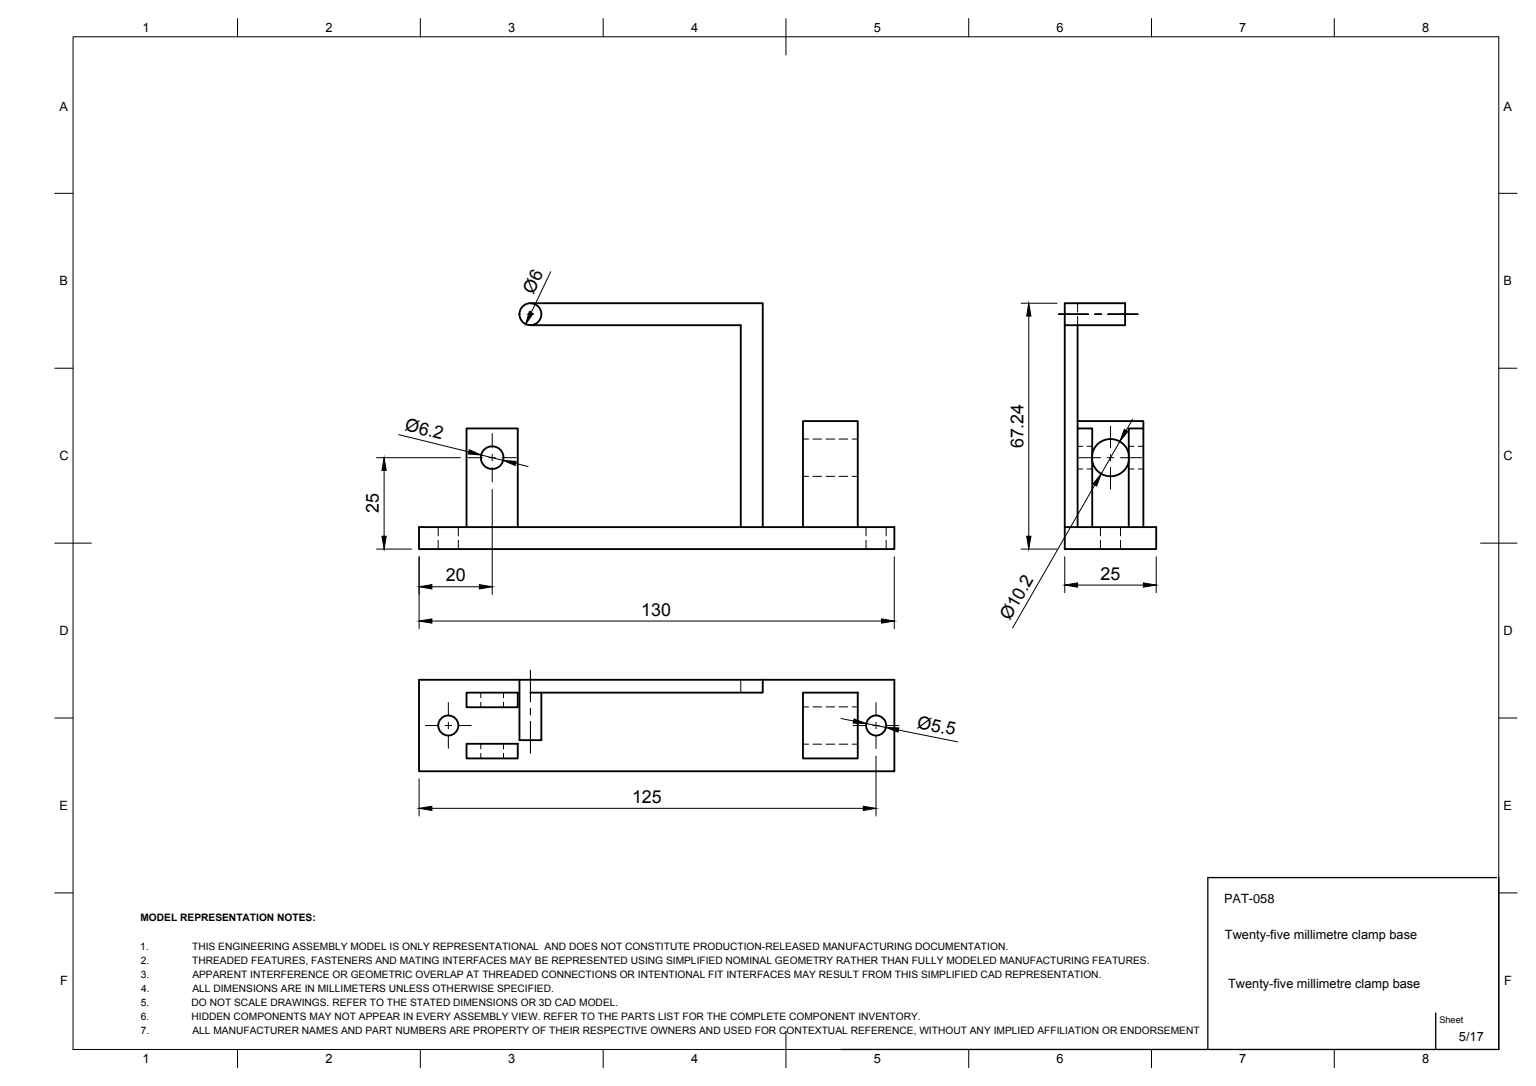
ISO-10303-21;
HEADER;
/* Generated by software containing ST-Developer
 * from STEP Tools, Inc. (www.steptools.com) 
 */

FILE_DESCRIPTION(
/* description */ ('Horizontal push-pull toggle clamp'),
/* implementation_level */ '2;1');

FILE_NAME(
/* name */ 'Twenty-five millimetre clamp base.step',
/* time_stamp */ '2026-10-27T21:21:09-07:00',
/* author */ (''),
/* organization */ (''),
/* preprocessor_version */ 'ST-DEVELOPER v20.2',
/* originating_system */ 'Autodesk Translation Framework v15.17.0.0',
/* authorisation */ '');

FILE_SCHEMA (('AUTOMOTIVE_DESIGN { 1 0 10303 214 3 1 1 }'));
ENDSEC;

DATA;
#10=MECHANICAL_DESIGN_GEOMETRIC_PRESENTATION_REPRESENTATION('',(#185),#4791);
#159=SHAPE_REPRESENTATION_RELATIONSHIP('SRR','None',#4862,#172);
#172=ADVANCED_BREP_SHAPE_REPRESENTATION('',(#198),#4775);
#185=STYLED_ITEM('',(#5002),#198);
#198=MANIFOLD_SOLID_BREP('Body1',#2629);
#210=FACE_BOUND('',#522,.T.);
#211=FACE_BOUND('',#523,.T.);
#212=FACE_BOUND('',#524,.T.);
#213=FACE_BOUND('',#525,.T.);
#214=FACE_BOUND('',#526,.T.);
#215=FACE_BOUND('',#532,.T.);
#216=FACE_BOUND('',#534,.T.);
#217=FACE_BOUND('',#540,.T.);
#218=FACE_BOUND('',#545,.T.);
#219=FACE_BOUND('',#547,.T.);
#220=FACE_BOUND('',#552,.T.);
#221=FACE_BOUND('',#557,.T.);
#222=FACE_BOUND('',#558,.T.);
#256=PLANE('',#2795);
#257=PLANE('',#2796);
#258=PLANE('',#2797);
#259=PLANE('',#2798);
#260=PLANE('',#2799);
#261=PLANE('',#2800);
#262=PLANE('',#2801);
#263=PLANE('',#2802);
#264=PLANE('',#2812);
#265=PLANE('',#2813);
#266=PLANE('',#2814);
#267=PLANE('',#2815);
#268=PLANE('',#2816);
#269=PLANE('',#2823);
#270=PLANE('',#2824);
#271=PLANE('',#2825);
#272=PLANE('',#2826);
#273=PLANE('',#2827);
#274=PLANE('',#2828);
#275=PLANE('',#2829);
#276=PLANE('',#2830);
#277=PLANE('',#2831);
#278=PLANE('',#2832);
#279=PLANE('',#2833);
#280=PLANE('',#2834);
#281=PLANE('',#2835);
#282=PLANE('',#2836);
#362=FACE_OUTER_BOUND('',#513,.T.);
#363=FACE_OUTER_BOUND('',#514,.T.);
#364=FACE_OUTER_BOUND('',#515,.T.);
#365=FACE_OUTER_BOUND('',#516,.T.);
#366=FACE_OUTER_BOUND('',#517,.T.);
#367=FACE_OUTER_BOUND('',#518,.T.);
#368=FACE_OUTER_BOUND('',#519,.T.);
#369=FACE_OUTER_BOUND('',#520,.T.);
#370=FACE_OUTER_BOUND('',#521,.T.);
#371=FACE_OUTER_BOUND('',#527,.T.);
#372=FACE_OUTER_BOUND('',#528,.T.);
#373=FACE_OUTER_BOUND('',#529,.T.);
#374=FACE_OUTER_BOUND('',#530,.T.);
#375=FACE_OUTER_BOUND('',#531,.T.);
#376=FACE_OUTER_BOUND('',#533,.T.);
#377=FACE_OUTER_BOUND('',#535,.T.);
#378=FACE_OUTER_BOUND('',#536,.T.);
#379=FACE_OUTER_BOUND('',#537,.T.);
#380=FACE_OUTER_BOUND('',#538,.T.);
#381=FACE_OUTER_BOUND('',#539,.T.);
#382=FACE_OUTER_BOUND('',#541,.T.);
#383=FACE_OUTER_BOUND('',#542,.T.);
#384=FACE_OUTER_BOUND('',#543,.T.);
#385=FACE_OUTER_BOUND('',#544,.T.);
#386=FACE_OUTER_BOUND('',#546,.T.);
#387=FACE_OUTER_BOUND('',#548,.T.);
#388=FACE_OUTER_BOUND('',#549,.T.);
#389=FACE_OUTER_BOUND('',#550,.T.);
#390=FACE_OUTER_BOUND('',#551,.T.);
#391=FACE_OUTER_BOUND('',#553,.T.);
#392=FACE_OUTER_BOUND('',#554,.T.);
#393=FACE_OUTER_BOUND('',#555,.T.);
#394=FACE_OUTER_BOUND('',#556,.T.);
#513=EDGE_LOOP('',(#1783,#1784,#1785,#1786,#1787,#1788,#1789,#1790));
#514=EDGE_LOOP('',(#1791));
#515=EDGE_LOOP('',(#1792,#1793,#1794,#1795,#1796,#1797,#1798,#1799,#1800,
#1801,#1802));
#516=EDGE_LOOP('',(#1803,#1804,#1805,#1806));
#517=EDGE_LOOP('',(#1807,#1808,#1809,#1810));
#518=EDGE_LOOP('',(#1811,#1812,#1813,#1814));
#519=EDGE_LOOP('',(#1815,#1816,#1817,#1818));
#520=EDGE_LOOP('',(#1819,#1820,#1821,#1822,#1823,#1824));
#521=EDGE_LOOP('',(#1825,#1826,#1827,#1828,#1829,#1830,#1831,#1832));
#522=EDGE_LOOP('',(#1833,#1834,#1835,#1836));
#523=EDGE_LOOP('',(#1837,#1838,#1839,#1840));
#524=EDGE_LOOP('',(#1841,#1842,#1843,#1844));
#525=EDGE_LOOP('',(#1845));
#526=EDGE_LOOP('',(#1846));
#527=EDGE_LOOP('',(#1847,#1848,#1849,#1850));
#528=EDGE_LOOP('',(#1851,#1852,#1853,#1854));
#529=EDGE_LOOP('',(#1855,#1856,#1857,#1858));
#530=EDGE_LOOP('',(#1859,#1860,#1861,#1862));
#531=EDGE_LOOP('',(#1863,#1864,#1865,#1866));
#532=EDGE_LOOP('',(#1867));
#533=EDGE_LOOP('',(#1868,#1869,#1870,#1871));
#534=EDGE_LOOP('',(#1872));
#535=EDGE_LOOP('',(#1873,#1874,#1875,#1876));
#536=EDGE_LOOP('',(#1877,#1878,#1879,#1880));
#537=EDGE_LOOP('',(#1881,#1882,#1883,#1884));
#538=EDGE_LOOP('',(#1885,#1886,#1887,#1888));
#539=EDGE_LOOP('',(#1889,#1890,#1891,#1892));
#540=EDGE_LOOP('',(#1893));
#541=EDGE_LOOP('',(#1894,#1895,#1896,#1897));
#542=EDGE_LOOP('',(#1898,#1899,#1900,#1901));
#543=EDGE_LOOP('',(#1902,#1903,#1904,#1905));
#544=EDGE_LOOP('',(#1906,#1907,#1908,#1909));
#545=EDGE_LOOP('',(#1910));
#546=EDGE_LOOP('',(#1911,#1912,#1913,#1914));
#547=EDGE_LOOP('',(#1915));
#548=EDGE_LOOP('',(#1916,#1917,#1918,#1919));
#549=EDGE_LOOP('',(#1920,#1921,#1922,#1923));
#550=EDGE_LOOP('',(#1924,#1925,#1926,#1927));
#551=EDGE_LOOP('',(#1928,#1929,#1930,#1931));
#552=EDGE_LOOP('',(#1932));
#553=EDGE_LOOP('',(#1933,#1934,#1935,#1936));
#554=EDGE_LOOP('',(#1937,#1938,#1939,#1940));
#555=EDGE_LOOP('',(#1941,#1942,#1943,#1944));
#556=EDGE_LOOP('',(#1945,#1946,#1947,#1948));
#557=EDGE_LOOP('',(#1949));
#558=EDGE_LOOP('',(#1950));
#710=CIRCLE('',#2791,0.3);
#711=CIRCLE('',#2792,0.3);
#712=CIRCLE('',#2793,0.3);
#713=CIRCLE('',#2794,0.3);
#714=CIRCLE('',#2803,0.275);
#715=CIRCLE('',#2804,0.275);
#716=CIRCLE('',#2806,0.275);
#717=CIRCLE('',#2808,0.275);
#718=CIRCLE('',#2810,0.51);
#719=CIRCLE('',#2811,0.51);
#720=CIRCLE('',#2818,0.31);
#721=CIRCLE('',#2819,0.31);
#722=CIRCLE('',#2821,0.31);
#723=CIRCLE('',#2822,0.31);
#796=LINE('',#3862,#1016);
#797=LINE('',#3866,#1017);
#798=LINE('',#3870,#1018);
#799=LINE('',#3876,#1019);
#800=LINE('',#3878,#1020);
#801=LINE('',#3880,#1021);
#802=LINE('',#3882,#1022);
#803=LINE('',#3884,#1023);
#804=LINE('',#3886,#1024);
#805=LINE('',#3888,#1025);
#806=LINE('',#3890,#1026);
#807=LINE('',#3891,#1027);
#808=LINE('',#3894,#1028);
#809=LINE('',#3895,#1029);
#810=LINE('',#3898,#1030);
#811=LINE('',#3899,#1031);
#812=LINE('',#3902,#1032);
#813=LINE('',#3903,#1033);
#814=LINE('',#3906,#1034);
#815=LINE('',#3907,#1035);
#816=LINE('',#3909,#1036);
#817=LINE('',#3912,#1037);
#818=LINE('',#3914,#1038);
#819=LINE('',#3915,#1039);
#820=LINE('',#3918,#1040);
#821=LINE('',#3920,#1041);
#822=LINE('',#3922,#1042);
#823=LINE('',#3923,#1043);
#824=LINE('',#3926,#1044);
#825=LINE('',#3928,#1045);
#826=LINE('',#3930,#1046);
#827=LINE('',#3931,#1047);
#828=LINE('',#3934,#1048);
#829=LINE('',#3936,#1049);
#830=LINE('',#3938,#1050);
#831=LINE('',#3939,#1051);
#832=LINE('',#3947,#1052);
#833=LINE('',#3951,#1053);
#834=LINE('',#3956,#1054);
#835=LINE('',#3960,#1055);
#836=LINE('',#3962,#1056);
#837=LINE('',#3963,#1057);
#838=LINE('',#3966,#1058);
#839=LINE('',#3967,#1059);
#840=LINE('',#3970,#1060);
#841=LINE('',#3971,#1061);
#842=LINE('',#3973,#1062);
#843=LINE('',#3979,#1063);
#844=LINE('',#3985,#1064);
#845=LINE('',#3989,#1065);
#846=LINE('',#3991,#1066);
#847=LINE('',#3992,#1067);
#848=LINE('',#3995,#1068);
#849=LINE('',#3996,#1069);
#850=LINE('',#3999,#1070);
#851=LINE('',#4000,#1071);
#852=LINE('',#4002,#1072);
#853=LINE('',#4006,#1073);
#854=LINE('',#4008,#1074);
#855=LINE('',#4009,#1075);
#856=LINE('',#4012,#1076);
#857=LINE('',#4013,#1077);
#858=LINE('',#4016,#1078);
#859=LINE('',#4017,#1079);
#860=LINE('',#4019,#1080);
#861=LINE('',#4023,#1081);
#862=LINE('',#4024,#1082);
#863=LINE('',#4027,#1083);
#864=LINE('',#4028,#1084);
#865=LINE('',#4030,#1085);
#1016=VECTOR('',#3078,1.);
#1017=VECTOR('',#3081,1.);
#1018=VECTOR('',#3084,0.3);
#1019=VECTOR('',#3093,1.);
#1020=VECTOR('',#3094,1.);
#1021=VECTOR('',#3095,1.);
#1022=VECTOR('',#3096,1.);
#1023=VECTOR('',#3097,1.);
#1024=VECTOR('',#3098,1.);
#1025=VECTOR('',#3099,1.);
#1026=VECTOR('',#3100,1.);
#1027=VECTOR('',#3101,1.);
#1028=VECTOR('',#3104,1.);
#1029=VECTOR('',#3105,1.);
#1030=VECTOR('',#3108,1.);
#1031=VECTOR('',#3109,1.);
#1032=VECTOR('',#3112,1.);
#1033=VECTOR('',#3113,1.);
#1034=VECTOR('',#3116,1.);
#1035=VECTOR('',#3117,1.);
#1036=VECTOR('',#3120,1.);
#1037=VECTOR('',#3123,1.);
#1038=VECTOR('',#3124,1.);
#1039=VECTOR('',#3125,1.);
#1040=VECTOR('',#3126,1.);
#1041=VECTOR('',#3127,1.);
#1042=VECTOR('',#3128,1.);
#1043=VECTOR('',#3129,1.);
#1044=VECTOR('',#3130,1.);
#1045=VECTOR('',#3131,1.);
#1046=VECTOR('',#3132,1.);
#1047=VECTOR('',#3133,1.);
#1048=VECTOR('',#3134,1.);
#1049=VECTOR('',#3135,1.);
#1050=VECTOR('',#3136,1.);
#1051=VECTOR('',#3137,1.);
#1052=VECTOR('',#3146,0.275);
#1053=VECTOR('',#3151,0.275);
#1054=VECTOR('',#3156,0.51);
#1055=VECTOR('',#3161,1.);
#1056=VECTOR('',#3162,1.);
#1057=VECTOR('',#3163,1.);
#1058=VECTOR('',#3166,1.);
#1059=VECTOR('',#3167,1.);
#1060=VECTOR('',#3170,1.);
#1061=VECTOR('',#3171,1.);
#1062=VECTOR('',#3174,1.);
#1063=VECTOR('',#3181,0.31);
#1064=VECTOR('',#3188,0.31);
#1065=VECTOR('',#3193,1.);
#1066=VECTOR('',#3194,1.);
#1067=VECTOR('',#3195,1.);
#1068=VECTOR('',#3198,1.);
#1069=VECTOR('',#3199,1.);
#1070=VECTOR('',#3202,1.);
#1071=VECTOR('',#3203,1.);
#1072=VECTOR('',#3206,1.);
#1073=VECTOR('',#3211,1.);
#1074=VECTOR('',#3212,1.);
#1075=VECTOR('',#3213,1.);
#1076=VECTOR('',#3216,1.);
#1077=VECTOR('',#3217,1.);
#1078=VECTOR('',#3220,1.);
#1079=VECTOR('',#3221,1.);
#1080=VECTOR('',#3224,1.);
#1081=VECTOR('',#3229,1.);
#1082=VECTOR('',#3230,1.);
#1083=VECTOR('',#3233,1.);
#1084=VECTOR('',#3234,1.);
#1085=VECTOR('',#3237,1.);
#1236=VERTEX_POINT('',#3860);
#1237=VERTEX_POINT('',#3861);
#1238=VERTEX_POINT('',#3863);
#1239=VERTEX_POINT('',#3865);
#1240=VERTEX_POINT('',#3867);
#1241=VERTEX_POINT('',#3869);
#1242=VERTEX_POINT('',#3875);
#1243=VERTEX_POINT('',#3877);
#1244=VERTEX_POINT('',#3879);
#1245=VERTEX_POINT('',#3881);
#1246=VERTEX_POINT('',#3883);
#1247=VERTEX_POINT('',#3885);
#1248=VERTEX_POINT('',#3887);
#1249=VERTEX_POINT('',#3889);
#1250=VERTEX_POINT('',#3893);
#1251=VERTEX_POINT('',#3897);
#1252=VERTEX_POINT('',#3901);
#1253=VERTEX_POINT('',#3905);
#1254=VERTEX_POINT('',#3911);
#1255=VERTEX_POINT('',#3913);
#1256=VERTEX_POINT('',#3916);
#1257=VERTEX_POINT('',#3917);
#1258=VERTEX_POINT('',#3919);
#1259=VERTEX_POINT('',#3921);
#1260=VERTEX_POINT('',#3924);
#1261=VERTEX_POINT('',#3925);
#1262=VERTEX_POINT('',#3927);
#1263=VERTEX_POINT('',#3929);
#1264=VERTEX_POINT('',#3932);
#1265=VERTEX_POINT('',#3933);
#1266=VERTEX_POINT('',#3935);
#1267=VERTEX_POINT('',#3937);
#1268=VERTEX_POINT('',#3940);
#1269=VERTEX_POINT('',#3942);
#1270=VERTEX_POINT('',#3945);
#1271=VERTEX_POINT('',#3949);
#1272=VERTEX_POINT('',#3953);
#1273=VERTEX_POINT('',#3955);
#1274=VERTEX_POINT('',#3959);
#1275=VERTEX_POINT('',#3961);
#1276=VERTEX_POINT('',#3965);
#1277=VERTEX_POINT('',#3969);
#1278=VERTEX_POINT('',#3976);
#1279=VERTEX_POINT('',#3978);
#1280=VERTEX_POINT('',#3982);
#1281=VERTEX_POINT('',#3984);
#1282=VERTEX_POINT('',#3988);
#1283=VERTEX_POINT('',#3990);
#1284=VERTEX_POINT('',#3994);
#1285=VERTEX_POINT('',#3998);
#1286=VERTEX_POINT('',#4005);
#1287=VERTEX_POINT('',#4007);
#1288=VERTEX_POINT('',#4011);
#1289=VERTEX_POINT('',#4015);
#1290=VERTEX_POINT('',#4022);
#1291=VERTEX_POINT('',#4026);
#1453=EDGE_CURVE('',#1236,#1237,#796,.T.);
#1454=EDGE_CURVE('',#1238,#1236,#710,.T.);
#1455=EDGE_CURVE('',#1238,#1239,#797,.T.);
#1456=EDGE_CURVE('',#1240,#1239,#711,.T.);
#1457=EDGE_CURVE('',#1240,#1241,#798,.T.);
#1458=EDGE_CURVE('',#1241,#1241,#712,.T.);
#1459=EDGE_CURVE('',#1237,#1240,#713,.T.);
#1460=EDGE_CURVE('',#1239,#1242,#799,.T.);
#1461=EDGE_CURVE('',#1242,#1243,#800,.T.);
#1462=EDGE_CURVE('',#1244,#1243,#801,.T.);
#1463=EDGE_CURVE('',#1245,#1244,#802,.T.);
#1464=EDGE_CURVE('',#1245,#1246,#803,.T.);
#1465=EDGE_CURVE('',#1246,#1247,#804,.T.);
#1466=EDGE_CURVE('',#1248,#1247,#805,.T.);
#1467=EDGE_CURVE('',#1248,#1249,#806,.T.);
#1468=EDGE_CURVE('',#1249,#1237,#807,.T.);
#1469=EDGE_CURVE('',#1250,#1249,#808,.T.);
#1470=EDGE_CURVE('',#1236,#1250,#809,.T.);
#1471=EDGE_CURVE('',#1251,#1238,#810,.T.);
#1472=EDGE_CURVE('',#1251,#1242,#811,.T.);
#1473=EDGE_CURVE('',#1252,#1251,#812,.T.);
#1474=EDGE_CURVE('',#1243,#1252,#813,.T.);
#1475=EDGE_CURVE('',#1253,#1248,#814,.T.);
#1476=EDGE_CURVE('',#1250,#1253,#815,.T.);
#1477=EDGE_CURVE('',#1252,#1253,#816,.T.);
#1478=EDGE_CURVE('',#1247,#1254,#817,.T.);
#1479=EDGE_CURVE('',#1254,#1255,#818,.T.);
#1480=EDGE_CURVE('',#1255,#1244,#819,.T.);
#1481=EDGE_CURVE('',#1256,#1257,#820,.T.);
#1482=EDGE_CURVE('',#1257,#1258,#821,.T.);
#1483=EDGE_CURVE('',#1258,#1259,#822,.T.);
#1484=EDGE_CURVE('',#1259,#1256,#823,.T.);
#1485=EDGE_CURVE('',#1260,#1261,#824,.T.);
#1486=EDGE_CURVE('',#1261,#1262,#825,.T.);
#1487=EDGE_CURVE('',#1262,#1263,#826,.T.);
#1488=EDGE_CURVE('',#1263,#1260,#827,.T.);
#1489=EDGE_CURVE('',#1264,#1265,#828,.T.);
#1490=EDGE_CURVE('',#1265,#1266,#829,.T.);
#1491=EDGE_CURVE('',#1266,#1267,#830,.T.);
#1492=EDGE_CURVE('',#1267,#1264,#831,.T.);
#1493=EDGE_CURVE('',#1268,#1268,#714,.T.);
#1494=EDGE_CURVE('',#1269,#1269,#715,.T.);
#1495=EDGE_CURVE('',#1270,#1270,#716,.T.);
#1496=EDGE_CURVE('',#1270,#1269,#832,.T.);
#1497=EDGE_CURVE('',#1271,#1271,#717,.T.);
#1498=EDGE_CURVE('',#1271,#1268,#833,.T.);
#1499=EDGE_CURVE('',#1272,#1272,#718,.T.);
#1500=EDGE_CURVE('',#1272,#1273,#834,.T.);
#1501=EDGE_CURVE('',#1273,#1273,#719,.T.);
#1502=EDGE_CURVE('',#1265,#1274,#835,.T.);
#1503=EDGE_CURVE('',#1274,#1275,#836,.T.);
#1504=EDGE_CURVE('',#1275,#1266,#837,.T.);
#1505=EDGE_CURVE('',#1276,#1264,#838,.T.);
#1506=EDGE_CURVE('',#1274,#1276,#839,.T.);
#1507=EDGE_CURVE('',#1275,#1277,#840,.T.);
#1508=EDGE_CURVE('',#1267,#1277,#841,.T.);
#1509=EDGE_CURVE('',#1277,#1276,#842,.T.);
#1510=EDGE_CURVE('',#1278,#1278,#720,.T.);
#1511=EDGE_CURVE('',#1278,#1279,#843,.T.);
#1512=EDGE_CURVE('',#1279,#1279,#721,.T.);
#1513=EDGE_CURVE('',#1280,#1280,#722,.T.);
#1514=EDGE_CURVE('',#1280,#1281,#844,.T.);
#1515=EDGE_CURVE('',#1281,#1281,#723,.T.);
#1516=EDGE_CURVE('',#1261,#1282,#845,.T.);
#1517=EDGE_CURVE('',#1282,#1283,#846,.T.);
#1518=EDGE_CURVE('',#1283,#1262,#847,.T.);
#1519=EDGE_CURVE('',#1284,#1260,#848,.T.);
#1520=EDGE_CURVE('',#1282,#1284,#849,.T.);
#1521=EDGE_CURVE('',#1283,#1285,#850,.T.);
#1522=EDGE_CURVE('',#1263,#1285,#851,.T.);
#1523=EDGE_CURVE('',#1285,#1284,#852,.T.);
#1524=EDGE_CURVE('',#1257,#1286,#853,.T.);
#1525=EDGE_CURVE('',#1286,#1287,#854,.T.);
#1526=EDGE_CURVE('',#1287,#1258,#855,.T.);
#1527=EDGE_CURVE('',#1288,#1256,#856,.T.);
#1528=EDGE_CURVE('',#1286,#1288,#857,.T.);
#1529=EDGE_CURVE('',#1287,#1289,#858,.T.);
#1530=EDGE_CURVE('',#1259,#1289,#859,.T.);
#1531=EDGE_CURVE('',#1289,#1288,#860,.T.);
#1532=EDGE_CURVE('',#1290,#1245,#861,.T.);
#1533=EDGE_CURVE('',#1290,#1255,#862,.T.);
#1534=EDGE_CURVE('',#1291,#1290,#863,.T.);
#1535=EDGE_CURVE('',#1291,#1254,#864,.T.);
#1536=EDGE_CURVE('',#1246,#1291,#865,.T.);
#1783=ORIENTED_EDGE('',*,*,#1453,.F.);
#1784=ORIENTED_EDGE('',*,*,#1454,.F.);
#1785=ORIENTED_EDGE('',*,*,#1455,.T.);
#1786=ORIENTED_EDGE('',*,*,#1456,.F.);
#1787=ORIENTED_EDGE('',*,*,#1457,.T.);
#1788=ORIENTED_EDGE('',*,*,#1458,.T.);
#1789=ORIENTED_EDGE('',*,*,#1457,.F.);
#1790=ORIENTED_EDGE('',*,*,#1459,.F.);
#1791=ORIENTED_EDGE('',*,*,#1458,.F.);
#1792=ORIENTED_EDGE('',*,*,#1460,.T.);
#1793=ORIENTED_EDGE('',*,*,#1461,.T.);
#1794=ORIENTED_EDGE('',*,*,#1462,.F.);
#1795=ORIENTED_EDGE('',*,*,#1463,.F.);
#1796=ORIENTED_EDGE('',*,*,#1464,.T.);
#1797=ORIENTED_EDGE('',*,*,#1465,.T.);
#1798=ORIENTED_EDGE('',*,*,#1466,.F.);
#1799=ORIENTED_EDGE('',*,*,#1467,.T.);
#1800=ORIENTED_EDGE('',*,*,#1468,.T.);
#1801=ORIENTED_EDGE('',*,*,#1459,.T.);
#1802=ORIENTED_EDGE('',*,*,#1456,.T.);
#1803=ORIENTED_EDGE('',*,*,#1469,.F.);
#1804=ORIENTED_EDGE('',*,*,#1470,.F.);
#1805=ORIENTED_EDGE('',*,*,#1453,.T.);
#1806=ORIENTED_EDGE('',*,*,#1468,.F.);
#1807=ORIENTED_EDGE('',*,*,#1471,.F.);
#1808=ORIENTED_EDGE('',*,*,#1472,.T.);
#1809=ORIENTED_EDGE('',*,*,#1460,.F.);
#1810=ORIENTED_EDGE('',*,*,#1455,.F.);
#1811=ORIENTED_EDGE('',*,*,#1473,.F.);
#1812=ORIENTED_EDGE('',*,*,#1474,.F.);
#1813=ORIENTED_EDGE('',*,*,#1461,.F.);
#1814=ORIENTED_EDGE('',*,*,#1472,.F.);
#1815=ORIENTED_EDGE('',*,*,#1469,.T.);
#1816=ORIENTED_EDGE('',*,*,#1467,.F.);
#1817=ORIENTED_EDGE('',*,*,#1475,.F.);
#1818=ORIENTED_EDGE('',*,*,#1476,.F.);
#1819=ORIENTED_EDGE('',*,*,#1454,.T.);
#1820=ORIENTED_EDGE('',*,*,#1470,.T.);
#1821=ORIENTED_EDGE('',*,*,#1476,.T.);
#1822=ORIENTED_EDGE('',*,*,#1477,.F.);
#1823=ORIENTED_EDGE('',*,*,#1473,.T.);
#1824=ORIENTED_EDGE('',*,*,#1471,.T.);
#1825=ORIENTED_EDGE('',*,*,#1474,.T.);
#1826=ORIENTED_EDGE('',*,*,#1477,.T.);
#1827=ORIENTED_EDGE('',*,*,#1475,.T.);
#1828=ORIENTED_EDGE('',*,*,#1466,.T.);
#1829=ORIENTED_EDGE('',*,*,#1478,.T.);
#1830=ORIENTED_EDGE('',*,*,#1479,.T.);
#1831=ORIENTED_EDGE('',*,*,#1480,.T.);
#1832=ORIENTED_EDGE('',*,*,#1462,.T.);
#1833=ORIENTED_EDGE('',*,*,#1481,.T.);
#1834=ORIENTED_EDGE('',*,*,#1482,.T.);
#1835=ORIENTED_EDGE('',*,*,#1483,.T.);
#1836=ORIENTED_EDGE('',*,*,#1484,.T.);
#1837=ORIENTED_EDGE('',*,*,#1485,.T.);
#1838=ORIENTED_EDGE('',*,*,#1486,.T.);
#1839=ORIENTED_EDGE('',*,*,#1487,.T.);
#1840=ORIENTED_EDGE('',*,*,#1488,.T.);
#1841=ORIENTED_EDGE('',*,*,#1489,.T.);
#1842=ORIENTED_EDGE('',*,*,#1490,.T.);
#1843=ORIENTED_EDGE('',*,*,#1491,.T.);
#1844=ORIENTED_EDGE('',*,*,#1492,.T.);
#1845=ORIENTED_EDGE('',*,*,#1493,.T.);
#1846=ORIENTED_EDGE('',*,*,#1494,.T.);
#1847=ORIENTED_EDGE('',*,*,#1495,.F.);
#1848=ORIENTED_EDGE('',*,*,#1496,.T.);
#1849=ORIENTED_EDGE('',*,*,#1494,.F.);
#1850=ORIENTED_EDGE('',*,*,#1496,.F.);
#1851=ORIENTED_EDGE('',*,*,#1497,.F.);
#1852=ORIENTED_EDGE('',*,*,#1498,.T.);
#1853=ORIENTED_EDGE('',*,*,#1493,.F.);
#1854=ORIENTED_EDGE('',*,*,#1498,.F.);
#1855=ORIENTED_EDGE('',*,*,#1499,.F.);
#1856=ORIENTED_EDGE('',*,*,#1500,.T.);
#1857=ORIENTED_EDGE('',*,*,#1501,.F.);
#1858=ORIENTED_EDGE('',*,*,#1500,.F.);
#1859=ORIENTED_EDGE('',*,*,#1490,.F.);
#1860=ORIENTED_EDGE('',*,*,#1502,.T.);
#1861=ORIENTED_EDGE('',*,*,#1503,.T.);
#1862=ORIENTED_EDGE('',*,*,#1504,.T.);
#1863=ORIENTED_EDGE('',*,*,#1489,.F.);
#1864=ORIENTED_EDGE('',*,*,#1505,.F.);
#1865=ORIENTED_EDGE('',*,*,#1506,.F.);
#1866=ORIENTED_EDGE('',*,*,#1502,.F.);
#1867=ORIENTED_EDGE('',*,*,#1501,.T.);
#1868=ORIENTED_EDGE('',*,*,#1491,.F.);
#1869=ORIENTED_EDGE('',*,*,#1504,.F.);
#1870=ORIENTED_EDGE('',*,*,#1507,.T.);
#1871=ORIENTED_EDGE('',*,*,#1508,.F.);
#1872=ORIENTED_EDGE('',*,*,#1499,.T.);
#1873=ORIENTED_EDGE('',*,*,#1503,.F.);
#1874=ORIENTED_EDGE('',*,*,#1506,.T.);
#1875=ORIENTED_EDGE('',*,*,#1509,.F.);
#1876=ORIENTED_EDGE('',*,*,#1507,.F.);
#1877=ORIENTED_EDGE('',*,*,#1492,.F.);
#1878=ORIENTED_EDGE('',*,*,#1508,.T.);
#1879=ORIENTED_EDGE('',*,*,#1509,.T.);
#1880=ORIENTED_EDGE('',*,*,#1505,.T.);
#1881=ORIENTED_EDGE('',*,*,#1510,.F.);
#1882=ORIENTED_EDGE('',*,*,#1511,.T.);
#1883=ORIENTED_EDGE('',*,*,#1512,.F.);
#1884=ORIENTED_EDGE('',*,*,#1511,.F.);
#1885=ORIENTED_EDGE('',*,*,#1513,.F.);
#1886=ORIENTED_EDGE('',*,*,#1514,.T.);
#1887=ORIENTED_EDGE('',*,*,#1515,.F.);
#1888=ORIENTED_EDGE('',*,*,#1514,.F.);
#1889=ORIENTED_EDGE('',*,*,#1486,.F.);
#1890=ORIENTED_EDGE('',*,*,#1516,.T.);
#1891=ORIENTED_EDGE('',*,*,#1517,.T.);
#1892=ORIENTED_EDGE('',*,*,#1518,.T.);
#1893=ORIENTED_EDGE('',*,*,#1513,.T.);
#1894=ORIENTED_EDGE('',*,*,#1485,.F.);
#1895=ORIENTED_EDGE('',*,*,#1519,.F.);
#1896=ORIENTED_EDGE('',*,*,#1520,.F.);
#1897=ORIENTED_EDGE('',*,*,#1516,.F.);
#1898=ORIENTED_EDGE('',*,*,#1487,.F.);
#1899=ORIENTED_EDGE('',*,*,#1518,.F.);
#1900=ORIENTED_EDGE('',*,*,#1521,.T.);
#1901=ORIENTED_EDGE('',*,*,#1522,.F.);
#1902=ORIENTED_EDGE('',*,*,#1517,.F.);
#1903=ORIENTED_EDGE('',*,*,#1520,.T.);
#1904=ORIENTED_EDGE('',*,*,#1523,.F.);
#1905=ORIENTED_EDGE('',*,*,#1521,.F.);
#1906=ORIENTED_EDGE('',*,*,#1488,.F.);
#1907=ORIENTED_EDGE('',*,*,#1522,.T.);
#1908=ORIENTED_EDGE('',*,*,#1523,.T.);
#1909=ORIENTED_EDGE('',*,*,#1519,.T.);
#1910=ORIENTED_EDGE('',*,*,#1515,.T.);
#1911=ORIENTED_EDGE('',*,*,#1482,.F.);
#1912=ORIENTED_EDGE('',*,*,#1524,.T.);
#1913=ORIENTED_EDGE('',*,*,#1525,.T.);
#1914=ORIENTED_EDGE('',*,*,#1526,.T.);
#1915=ORIENTED_EDGE('',*,*,#1510,.T.);
#1916=ORIENTED_EDGE('',*,*,#1481,.F.);
#1917=ORIENTED_EDGE('',*,*,#1527,.F.);
#1918=ORIENTED_EDGE('',*,*,#1528,.F.);
#1919=ORIENTED_EDGE('',*,*,#1524,.F.);
#1920=ORIENTED_EDGE('',*,*,#1483,.F.);
#1921=ORIENTED_EDGE('',*,*,#1526,.F.);
#1922=ORIENTED_EDGE('',*,*,#1529,.T.);
#1923=ORIENTED_EDGE('',*,*,#1530,.F.);
#1924=ORIENTED_EDGE('',*,*,#1525,.F.);
#1925=ORIENTED_EDGE('',*,*,#1528,.T.);
#1926=ORIENTED_EDGE('',*,*,#1531,.F.);
#1927=ORIENTED_EDGE('',*,*,#1529,.F.);
#1928=ORIENTED_EDGE('',*,*,#1484,.F.);
#1929=ORIENTED_EDGE('',*,*,#1530,.T.);
#1930=ORIENTED_EDGE('',*,*,#1531,.T.);
#1931=ORIENTED_EDGE('',*,*,#1527,.T.);
#1932=ORIENTED_EDGE('',*,*,#1512,.T.);
#1933=ORIENTED_EDGE('',*,*,#1532,.T.);
#1934=ORIENTED_EDGE('',*,*,#1463,.T.);
#1935=ORIENTED_EDGE('',*,*,#1480,.F.);
#1936=ORIENTED_EDGE('',*,*,#1533,.F.);
#1937=ORIENTED_EDGE('',*,*,#1534,.T.);
#1938=ORIENTED_EDGE('',*,*,#1533,.T.);
#1939=ORIENTED_EDGE('',*,*,#1479,.F.);
#1940=ORIENTED_EDGE('',*,*,#1535,.F.);
#1941=ORIENTED_EDGE('',*,*,#1536,.T.);
#1942=ORIENTED_EDGE('',*,*,#1535,.T.);
#1943=ORIENTED_EDGE('',*,*,#1478,.F.);
#1944=ORIENTED_EDGE('',*,*,#1465,.F.);
#1945=ORIENTED_EDGE('',*,*,#1536,.F.);
#1946=ORIENTED_EDGE('',*,*,#1464,.F.);
#1947=ORIENTED_EDGE('',*,*,#1532,.F.);
#1948=ORIENTED_EDGE('',*,*,#1534,.F.);
#1949=ORIENTED_EDGE('',*,*,#1495,.T.);
#1950=ORIENTED_EDGE('',*,*,#1497,.T.);
#2443=CYLINDRICAL_SURFACE('',#2790,0.3);
#2444=CYLINDRICAL_SURFACE('',#2805,0.275);
#2445=CYLINDRICAL_SURFACE('',#2807,0.275);
#2446=CYLINDRICAL_SURFACE('',#2809,0.51);
#2447=CYLINDRICAL_SURFACE('',#2817,0.31);
#2448=CYLINDRICAL_SURFACE('',#2820,0.31);
#2478=ADVANCED_FACE('',(#362),#2443,.T.);
#2479=ADVANCED_FACE('',(#363),#256,.F.);
#2480=ADVANCED_FACE('',(#364),#257,.T.);
#2481=ADVANCED_FACE('',(#365),#258,.T.);
#2482=ADVANCED_FACE('',(#366),#259,.T.);
#2483=ADVANCED_FACE('',(#367),#260,.T.);
#2484=ADVANCED_FACE('',(#368),#261,.T.);
#2485=ADVANCED_FACE('',(#369),#262,.F.);
#2486=ADVANCED_FACE('',(#370,#210,#211,#212,#213,#214),#263,.T.);
#2487=ADVANCED_FACE('',(#371),#2444,.F.);
#2488=ADVANCED_FACE('',(#372),#2445,.F.);
#2489=ADVANCED_FACE('',(#373),#2446,.F.);
#2490=ADVANCED_FACE('',(#374),#264,.F.);
#2491=ADVANCED_FACE('',(#375,#215),#265,.T.);
#2492=ADVANCED_FACE('',(#376,#216),#266,.T.);
#2493=ADVANCED_FACE('',(#377),#267,.T.);
#2494=ADVANCED_FACE('',(#378),#268,.T.);
#2495=ADVANCED_FACE('',(#379),#2447,.F.);
#2496=ADVANCED_FACE('',(#380),#2448,.F.);
#2497=ADVANCED_FACE('',(#381,#217),#269,.F.);
#2498=ADVANCED_FACE('',(#382),#270,.T.);
#2499=ADVANCED_FACE('',(#383),#271,.T.);
#2500=ADVANCED_FACE('',(#384),#272,.T.);
#2501=ADVANCED_FACE('',(#385,#218),#273,.T.);
#2502=ADVANCED_FACE('',(#386,#219),#274,.F.);
#2503=ADVANCED_FACE('',(#387),#275,.T.);
#2504=ADVANCED_FACE('',(#388),#276,.T.);
#2505=ADVANCED_FACE('',(#389),#277,.T.);
#2506=ADVANCED_FACE('',(#390,#220),#278,.T.);
#2507=ADVANCED_FACE('',(#391),#279,.T.);
#2508=ADVANCED_FACE('',(#392),#280,.T.);
#2509=ADVANCED_FACE('',(#393),#281,.T.);
#2510=ADVANCED_FACE('',(#394,#221,#222),#282,.F.);
#2629=CLOSED_SHELL('',(#2478,#2479,#2480,#2481,#2482,#2483,#2484,#2485,
#2486,#2487,#2488,#2489,#2490,#2491,#2492,#2493,#2494,#2495,#2496,#2497,
#2498,#2499,#2500,#2501,#2502,#2503,#2504,#2505,#2506,#2507,#2508,#2509,
#2510));
#2789=AXIS2_PLACEMENT_3D('',#3858,#3074,#3075);
#2790=AXIS2_PLACEMENT_3D('',#3859,#3076,#3077);
#2791=AXIS2_PLACEMENT_3D('',#3864,#3079,#3080);
#2792=AXIS2_PLACEMENT_3D('',#3868,#3082,#3083);
#2793=AXIS2_PLACEMENT_3D('',#3871,#3085,#3086);
#2794=AXIS2_PLACEMENT_3D('',#3872,#3087,#3088);
#2795=AXIS2_PLACEMENT_3D('',#3873,#3089,#3090);
#2796=AXIS2_PLACEMENT_3D('',#3874,#3091,#3092);
#2797=AXIS2_PLACEMENT_3D('',#3892,#3102,#3103);
#2798=AXIS2_PLACEMENT_3D('',#3896,#3106,#3107);
#2799=AXIS2_PLACEMENT_3D('',#3900,#3110,#3111);
#2800=AXIS2_PLACEMENT_3D('',#3904,#3114,#3115);
#2801=AXIS2_PLACEMENT_3D('',#3908,#3118,#3119);
#2802=AXIS2_PLACEMENT_3D('',#3910,#3121,#3122);
#2803=AXIS2_PLACEMENT_3D('',#3941,#3138,#3139);
#2804=AXIS2_PLACEMENT_3D('',#3943,#3140,#3141);
#2805=AXIS2_PLACEMENT_3D('',#3944,#3142,#3143);
#2806=AXIS2_PLACEMENT_3D('',#3946,#3144,#3145);
#2807=AXIS2_PLACEMENT_3D('',#3948,#3147,#3148);
#2808=AXIS2_PLACEMENT_3D('',#3950,#3149,#3150);
#2809=AXIS2_PLACEMENT_3D('',#3952,#3152,#3153);
#2810=AXIS2_PLACEMENT_3D('',#3954,#3154,#3155);
#2811=AXIS2_PLACEMENT_3D('',#3957,#3157,#3158);
#2812=AXIS2_PLACEMENT_3D('',#3958,#3159,#3160);
#2813=AXIS2_PLACEMENT_3D('',#3964,#3164,#3165);
#2814=AXIS2_PLACEMENT_3D('',#3968,#3168,#3169);
#2815=AXIS2_PLACEMENT_3D('',#3972,#3172,#3173);
#2816=AXIS2_PLACEMENT_3D('',#3974,#3175,#3176);
#2817=AXIS2_PLACEMENT_3D('',#3975,#3177,#3178);
#2818=AXIS2_PLACEMENT_3D('',#3977,#3179,#3180);
#2819=AXIS2_PLACEMENT_3D('',#3980,#3182,#3183);
#2820=AXIS2_PLACEMENT_3D('',#3981,#3184,#3185);
#2821=AXIS2_PLACEMENT_3D('',#3983,#3186,#3187);
#2822=AXIS2_PLACEMENT_3D('',#3986,#3189,#3190);
#2823=AXIS2_PLACEMENT_3D('',#3987,#3191,#3192);
#2824=AXIS2_PLACEMENT_3D('',#3993,#3196,#3197);
#2825=AXIS2_PLACEMENT_3D('',#3997,#3200,#3201);
#2826=AXIS2_PLACEMENT_3D('',#4001,#3204,#3205);
#2827=AXIS2_PLACEMENT_3D('',#4003,#3207,#3208);
#2828=AXIS2_PLACEMENT_3D('',#4004,#3209,#3210);
#2829=AXIS2_PLACEMENT_3D('',#4010,#3214,#3215);
#2830=AXIS2_PLACEMENT_3D('',#4014,#3218,#3219);
#2831=AXIS2_PLACEMENT_3D('',#4018,#3222,#3223);
#2832=AXIS2_PLACEMENT_3D('',#4020,#3225,#3226);
#2833=AXIS2_PLACEMENT_3D('',#4021,#3227,#3228);
#2834=AXIS2_PLACEMENT_3D('',#4025,#3231,#3232);
#2835=AXIS2_PLACEMENT_3D('',#4029,#3235,#3236);
#2836=AXIS2_PLACEMENT_3D('',#4031,#3238,#3239);
#3074=DIRECTION('axis',(0.,0.,1.));
#3075=DIRECTION('refdir',(1.,0.,0.));
#3076=DIRECTION('center_axis',(0.,1.,0.));
#3077=DIRECTION('ref_axis',(1.,0.,0.));
#3078=DIRECTION('',(0.,1.,0.));
#3079=DIRECTION('center_axis',(0.,1.,0.));
#3080=DIRECTION('ref_axis',(1.,0.,0.));
#3081=DIRECTION('',(0.,1.,0.));
#3082=DIRECTION('center_axis',(0.,1.,0.));
#3083=DIRECTION('ref_axis',(1.,0.,0.));
#3084=DIRECTION('',(0.,-1.,0.));
#3085=DIRECTION('center_axis',(0.,1.,0.));
#3086=DIRECTION('ref_axis',(1.,0.,0.));
#3087=DIRECTION('center_axis',(0.,1.,0.));
#3088=DIRECTION('ref_axis',(1.,0.,0.));
#3089=DIRECTION('center_axis',(0.,1.,0.));
#3090=DIRECTION('ref_axis',(1.,0.,0.));
#3091=DIRECTION('center_axis',(0.,1.,0.));
#3092=DIRECTION('ref_axis',(-1.,0.,0.));
#3093=DIRECTION('',(1.,0.,0.));
#3094=DIRECTION('',(0.,0.,-1.));
#3095=DIRECTION('',(-1.,0.,0.));
#3096=DIRECTION('',(0.,0.,1.));
#3097=DIRECTION('',(-1.,0.,0.));
#3098=DIRECTION('',(0.,0.,1.));
#3099=DIRECTION('',(-1.,0.,0.));
#3100=DIRECTION('',(0.,0.,1.));
#3101=DIRECTION('',(-1.,0.,0.));
#3102=DIRECTION('center_axis',(0.,0.,-1.));
#3103=DIRECTION('ref_axis',(-1.,0.,0.));
#3104=DIRECTION('',(0.,1.,0.));
#3105=DIRECTION('',(1.,0.,0.));
#3106=DIRECTION('center_axis',(0.,0.,1.));
#3107=DIRECTION('ref_axis',(1.,0.,0.));
#3108=DIRECTION('',(-1.,0.,0.));
#3109=DIRECTION('',(0.,1.,0.));
#3110=DIRECTION('center_axis',(1.,0.,0.));
#3111=DIRECTION('ref_axis',(0.,0.,-1.));
#3112=DIRECTION('',(0.,0.,1.));
#3113=DIRECTION('',(0.,-1.,0.));
#3114=DIRECTION('center_axis',(-1.,0.,0.));
#3115=DIRECTION('ref_axis',(0.,0.,1.));
#3116=DIRECTION('',(0.,1.,0.));
#3117=DIRECTION('',(0.,0.,-1.));
#3118=DIRECTION('center_axis',(0.,1.,0.));
#3119=DIRECTION('ref_axis',(1.,0.,0.));
#3120=DIRECTION('',(-1.,0.,0.));
#3121=DIRECTION('center_axis',(0.,0.,1.));
#3122=DIRECTION('ref_axis',(1.,0.,0.));
#3123=DIRECTION('',(0.,-1.,0.));
#3124=DIRECTION('',(1.,0.,0.));
#3125=DIRECTION('',(0.,1.,0.));
#3126=DIRECTION('',(0.,-1.,0.));
#3127=DIRECTION('',(-1.,0.,0.));
#3128=DIRECTION('',(0.,1.,0.));
#3129=DIRECTION('',(1.,0.,0.));
#3130=DIRECTION('',(0.,-1.,0.));
#3131=DIRECTION('',(-1.,0.,0.));
#3132=DIRECTION('',(0.,1.,0.));
#3133=DIRECTION('',(1.,0.,0.));
#3134=DIRECTION('',(0.,-1.,0.));
#3135=DIRECTION('',(-1.,0.,0.));
#3136=DIRECTION('',(0.,1.,0.));
#3137=DIRECTION('',(1.,0.,0.));
#3138=DIRECTION('center_axis',(0.,0.,-1.));
#3139=DIRECTION('ref_axis',(1.,0.,0.));
#3140=DIRECTION('center_axis',(0.,0.,-1.));
#3141=DIRECTION('ref_axis',(1.,0.,0.));
#3142=DIRECTION('center_axis',(0.,0.,1.));
#3143=DIRECTION('ref_axis',(1.,0.,0.));
#3144=DIRECTION('center_axis',(0.,0.,1.));
#3145=DIRECTION('ref_axis',(1.,0.,0.));
#3146=DIRECTION('',(0.,0.,1.));
#3147=DIRECTION('center_axis',(0.,0.,1.));
#3148=DIRECTION('ref_axis',(1.,0.,0.));
#3149=DIRECTION('center_axis',(0.,0.,1.));
#3150=DIRECTION('ref_axis',(1.,0.,0.));
#3151=DIRECTION('',(0.,0.,1.));
#3152=DIRECTION('center_axis',(1.,0.,0.));
#3153=DIRECTION('ref_axis',(0.,0.,-1.));
#3154=DIRECTION('center_axis',(1.,0.,0.));
#3155=DIRECTION('ref_axis',(0.,0.,-1.));
#3156=DIRECTION('',(1.,0.,0.));
#3157=DIRECTION('center_axis',(-1.,0.,0.));
#3158=DIRECTION('ref_axis',(0.,0.,-1.));
#3159=DIRECTION('center_axis',(0.,1.,0.));
#3160=DIRECTION('ref_axis',(1.,0.,0.));
#3161=DIRECTION('',(0.,0.,1.));
#3162=DIRECTION('',(-1.,0.,0.));
#3163=DIRECTION('',(0.,0.,-1.));
#3164=DIRECTION('center_axis',(1.,0.,0.));
#3165=DIRECTION('ref_axis',(0.,0.,-1.));
#3166=DIRECTION('',(0.,0.,-1.));
#3167=DIRECTION('',(0.,1.,0.));
#3168=DIRECTION('center_axis',(-1.,0.,0.));
#3169=DIRECTION('ref_axis',(0.,0.,1.));
#3170=DIRECTION('',(0.,1.,0.));
#3171=DIRECTION('',(0.,0.,1.));
#3172=DIRECTION('center_axis',(0.,0.,1.));
#3173=DIRECTION('ref_axis',(1.,0.,0.));
#3174=DIRECTION('',(1.,0.,0.));
#3175=DIRECTION('center_axis',(0.,1.,0.));
#3176=DIRECTION('ref_axis',(0.,0.,1.));
#3177=DIRECTION('center_axis',(0.,1.,0.));
#3178=DIRECTION('ref_axis',(1.,0.,0.));
#3179=DIRECTION('center_axis',(0.,1.,0.));
#3180=DIRECTION('ref_axis',(1.,0.,0.));
#3181=DIRECTION('',(0.,1.,0.));
#3182=DIRECTION('center_axis',(0.,-1.,0.));
#3183=DIRECTION('ref_axis',(1.,0.,0.));
#3184=DIRECTION('center_axis',(0.,1.,0.));
#3185=DIRECTION('ref_axis',(1.,0.,0.));
#3186=DIRECTION('center_axis',(0.,1.,0.));
#3187=DIRECTION('ref_axis',(1.,0.,0.));
#3188=DIRECTION('',(0.,1.,0.));
#3189=DIRECTION('center_axis',(0.,-1.,0.));
#3190=DIRECTION('ref_axis',(1.,0.,0.));
#3191=DIRECTION('center_axis',(0.,1.,0.));
#3192=DIRECTION('ref_axis',(1.,0.,0.));
#3193=DIRECTION('',(0.,0.,1.));
#3194=DIRECTION('',(-1.,0.,0.));
#3195=DIRECTION('',(0.,0.,-1.));
#3196=DIRECTION('center_axis',(1.,0.,0.));
#3197=DIRECTION('ref_axis',(0.,0.,-1.));
#3198=DIRECTION('',(0.,0.,-1.));
#3199=DIRECTION('',(0.,1.,0.));
#3200=DIRECTION('center_axis',(-1.,0.,0.));
#3201=DIRECTION('ref_axis',(0.,0.,1.));
#3202=DIRECTION('',(0.,1.,0.));
#3203=DIRECTION('',(0.,0.,1.));
#3204=DIRECTION('center_axis',(0.,0.,1.));
#3205=DIRECTION('ref_axis',(1.,0.,0.));
#3206=DIRECTION('',(1.,0.,0.));
#3207=DIRECTION('center_axis',(0.,1.,0.));
#3208=DIRECTION('ref_axis',(0.,0.,1.));
#3209=DIRECTION('center_axis',(0.,1.,0.));
#3210=DIRECTION('ref_axis',(1.,0.,0.));
#3211=DIRECTION('',(0.,0.,1.));
#3212=DIRECTION('',(-1.,0.,0.));
#3213=DIRECTION('',(0.,0.,-1.));
#3214=DIRECTION('center_axis',(1.,0.,0.));
#3215=DIRECTION('ref_axis',(0.,0.,-1.));
#3216=DIRECTION('',(0.,0.,-1.));
#3217=DIRECTION('',(0.,1.,0.));
#3218=DIRECTION('center_axis',(-1.,0.,0.));
#3219=DIRECTION('ref_axis',(0.,0.,1.));
#3220=DIRECTION('',(0.,1.,0.));
#3221=DIRECTION('',(0.,0.,1.));
#3222=DIRECTION('center_axis',(0.,0.,1.));
#3223=DIRECTION('ref_axis',(1.,0.,0.));
#3224=DIRECTION('',(1.,0.,0.));
#3225=DIRECTION('center_axis',(0.,1.,0.));
#3226=DIRECTION('ref_axis',(0.,0.,1.));
#3227=DIRECTION('center_axis',(1.,0.,0.));
#3228=DIRECTION('ref_axis',(0.,1.,0.));
#3229=DIRECTION('',(0.,1.,0.));
#3230=DIRECTION('',(0.,0.,1.));
#3231=DIRECTION('center_axis',(0.,-1.,0.));
#3232=DIRECTION('ref_axis',(1.,0.,0.));
#3233=DIRECTION('',(1.,0.,0.));
#3234=DIRECTION('',(0.,0.,1.));
#3235=DIRECTION('center_axis',(-1.,0.,0.));
#3236=DIRECTION('ref_axis',(0.,-1.,0.));
#3237=DIRECTION('',(0.,-1.,0.));
#3238=DIRECTION('center_axis',(0.,0.,1.));
#3239=DIRECTION('ref_axis',(1.,0.,0.));
#3858=CARTESIAN_POINT('',(0.,0.,0.));
#3859=CARTESIAN_POINT('Origin',(1.04595925965485,-0.4,6.42376977244362));
#3860=CARTESIAN_POINT('',(1.04595925965485,0.9,6.12376977244362));
#3861=CARTESIAN_POINT('',(1.04595925965485,1.25,6.12376977244362));
#3862=CARTESIAN_POINT('',(1.04595925965485,0.9,6.12376977244362));
#3863=CARTESIAN_POINT('',(1.04595925965485,0.9,6.72376977244362));
#3864=CARTESIAN_POINT('Origin',(1.04595925965485,0.9,6.42376977244362));
#3865=CARTESIAN_POINT('',(1.04595925965485,1.25,6.72376977244362));
#3866=CARTESIAN_POINT('',(1.04595925965485,0.9,6.72376977244362));
#3867=CARTESIAN_POINT('',(0.745959259654855,1.25,6.42376977244362));
#3868=CARTESIAN_POINT('Origin',(1.04595925965485,1.25,6.42376977244362));
#3869=CARTESIAN_POINT('',(0.745959259654855,-0.4,6.42376977244362));
#3870=CARTESIAN_POINT('',(0.745959259654855,-0.4,6.42376977244362));
#3871=CARTESIAN_POINT('Origin',(1.04595925965485,-0.4,6.42376977244362));
#3872=CARTESIAN_POINT('Origin',(1.04595925965485,1.25,6.42376977244362));
#3873=CARTESIAN_POINT('Origin',(1.04595925965485,-0.4,6.42376977244362));
#3874=CARTESIAN_POINT('Origin',(11.,1.25,0.));
#3875=CARTESIAN_POINT('',(7.4,1.25,6.72376977244362));
#3876=CARTESIAN_POINT('',(7.4,1.25,6.72376977244362));
#3877=CARTESIAN_POINT('',(7.4,1.25,0.6));
#3878=CARTESIAN_POINT('',(7.4,1.25,6.12376977244362));
#3879=CARTESIAN_POINT('',(11.,1.25,0.6));
#3880=CARTESIAN_POINT('',(11.,1.25,0.6));
#3881=CARTESIAN_POINT('',(11.,1.25,0.));
#3882=CARTESIAN_POINT('',(11.,1.25,0.));
#3883=CARTESIAN_POINT('',(-2.,1.25,0.));
#3884=CARTESIAN_POINT('',(11.,1.25,0.));
#3885=CARTESIAN_POINT('',(-2.,1.25,0.6));
#3886=CARTESIAN_POINT('',(-2.,1.25,0.));
#3887=CARTESIAN_POINT('',(6.8,1.25,0.6));
#3888=CARTESIAN_POINT('',(11.,1.25,0.6));
#3889=CARTESIAN_POINT('',(6.8,1.25,6.12376977244362));
#3890=CARTESIAN_POINT('',(6.8,1.25,6.42376977244362));
#3891=CARTESIAN_POINT('',(1.04595925965485,1.25,6.12376977244362));
#3892=CARTESIAN_POINT('Origin',(7.4,0.9,6.12376977244362));
#3893=CARTESIAN_POINT('',(6.8,0.9,6.12376977244362));
#3894=CARTESIAN_POINT('',(6.8,0.9,6.12376977244362));
#3895=CARTESIAN_POINT('',(1.04595925965485,0.9,6.12376977244362));
#3896=CARTESIAN_POINT('Origin',(1.04595925965485,0.9,6.72376977244362));
#3897=CARTESIAN_POINT('',(7.4,0.9,6.72376977244362));
#3898=CARTESIAN_POINT('',(7.4,0.9,6.72376977244362));
#3899=CARTESIAN_POINT('',(7.4,0.9,6.72376977244362));
#3900=CARTESIAN_POINT('Origin',(7.4,0.9,6.42376977244362));
#3901=CARTESIAN_POINT('',(7.4,0.9,0.6));
#3902=CARTESIAN_POINT('',(7.4,0.9,6.12376977244362));
#3903=CARTESIAN_POINT('',(7.4,0.45,0.6));
#3904=CARTESIAN_POINT('Origin',(6.8,0.9,0.5));
#3905=CARTESIAN_POINT('',(6.8,0.9,0.6));
#3906=CARTESIAN_POINT('',(6.8,0.45,0.6));
#3907=CARTESIAN_POINT('',(6.8,0.9,6.42376977244362));
#3908=CARTESIAN_POINT('Origin',(7.1,0.9,3.46188488622181));
#3909=CARTESIAN_POINT('',(5.8,0.9,0.6));
#3910=CARTESIAN_POINT('Origin',(4.5,0.,0.6));
#3911=CARTESIAN_POINT('',(-2.,-1.25,0.6));
#3912=CARTESIAN_POINT('',(-2.,1.25,0.6));
#3913=CARTESIAN_POINT('',(11.,-1.25,0.6));
#3914=CARTESIAN_POINT('',(-2.,-1.25,0.6));
#3915=CARTESIAN_POINT('',(11.,-1.25,0.6));
#3916=CARTESIAN_POINT('',(0.7,-0.5,0.6));
#3917=CARTESIAN_POINT('',(0.7,-0.9,0.6));
#3918=CARTESIAN_POINT('',(0.7,-0.45,0.6));
#3919=CARTESIAN_POINT('',(-0.7,-0.9,0.6));
#3920=CARTESIAN_POINT('',(2.25,-0.9,0.6));
#3921=CARTESIAN_POINT('',(-0.7,-0.5,0.6));
#3922=CARTESIAN_POINT('',(-0.7,-0.45,0.6));
#3923=CARTESIAN_POINT('',(2.25,-0.5,0.6));
#3924=CARTESIAN_POINT('',(0.7,0.9,0.6));
#3925=CARTESIAN_POINT('',(0.7,0.5,0.6));
#3926=CARTESIAN_POINT('',(0.7,0.25,0.6));
#3927=CARTESIAN_POINT('',(-0.7,0.5,0.6));
#3928=CARTESIAN_POINT('',(2.25,0.5,0.6));
#3929=CARTESIAN_POINT('',(-0.7,0.9,0.6));
#3930=CARTESIAN_POINT('',(-0.7,0.25,0.6));
#3931=CARTESIAN_POINT('',(2.25,0.9,0.6));
#3932=CARTESIAN_POINT('',(10.,0.9,0.6));
#3933=CARTESIAN_POINT('',(10.,-0.9,0.6));
#3934=CARTESIAN_POINT('',(10.,-0.45,0.6));
#3935=CARTESIAN_POINT('',(8.5,-0.9,0.6));
#3936=CARTESIAN_POINT('',(6.875,-0.9,0.6));
#3937=CARTESIAN_POINT('',(8.5,0.9,0.6));
#3938=CARTESIAN_POINT('',(8.5,-0.45,0.6));
#3939=CARTESIAN_POINT('',(6.875,0.9,0.6));
#3940=CARTESIAN_POINT('',(10.225,3.36777869765523E-17,0.6));
#3941=CARTESIAN_POINT('Origin',(10.5,0.,0.6));
#3942=CARTESIAN_POINT('',(-1.475,3.36777869765522E-17,0.6));
#3943=CARTESIAN_POINT('Origin',(-1.2,0.,0.6));
#3944=CARTESIAN_POINT('Origin',(-1.2,0.,-0.1));
#3945=CARTESIAN_POINT('',(-1.475,-3.36777869765522E-17,0.));
#3946=CARTESIAN_POINT('Origin',(-1.2,0.,0.));
#3947=CARTESIAN_POINT('',(-1.475,-3.36777869765522E-17,-0.1));
#3948=CARTESIAN_POINT('Origin',(10.5,0.,-0.1));
#3949=CARTESIAN_POINT('',(10.225,-3.36777869765523E-17,0.));
#3950=CARTESIAN_POINT('Origin',(10.5,0.,0.));
#3951=CARTESIAN_POINT('',(10.225,-3.36777869765523E-17,-0.1));
#3952=CARTESIAN_POINT('Origin',(8.4,0.,2.5));
#3953=CARTESIAN_POINT('',(8.5,-6.2456986756515E-17,3.01));
#3954=CARTESIAN_POINT('Origin',(8.5,0.,2.5));
#3955=CARTESIAN_POINT('',(10.,6.2456986756515E-17,3.01));
#3956=CARTESIAN_POINT('',(8.4,-6.2456986756515E-17,3.01));
#3957=CARTESIAN_POINT('Origin',(10.,0.,2.5));
#3958=CARTESIAN_POINT('Origin',(9.25,-0.9,2.));
#3959=CARTESIAN_POINT('',(10.,-0.9,3.5));
#3960=CARTESIAN_POINT('',(10.,-0.9,0.5));
#3961=CARTESIAN_POINT('',(8.5,-0.9,3.5));
#3962=CARTESIAN_POINT('',(10.,-0.9,3.5));
#3963=CARTESIAN_POINT('',(8.5,-0.9,3.5));
#3964=CARTESIAN_POINT('Origin',(10.,-0.9,3.5));
#3965=CARTESIAN_POINT('',(10.,0.9,3.5));
#3966=CARTESIAN_POINT('',(10.,0.9,0.5));
#3967=CARTESIAN_POINT('',(10.,-0.9,3.5));
#3968=CARTESIAN_POINT('Origin',(8.5,-0.9,0.5));
#3969=CARTESIAN_POINT('',(8.5,0.9,3.5));
#3970=CARTESIAN_POINT('',(8.5,-0.9,3.5));
#3971=CARTESIAN_POINT('',(8.5,0.9,3.5));
#3972=CARTESIAN_POINT('Origin',(8.5,-0.9,3.5));
#3973=CARTESIAN_POINT('',(10.,0.9,3.5));
#3974=CARTESIAN_POINT('Origin',(9.25,0.9,2.));
#3975=CARTESIAN_POINT('Origin',(0.,-1.,2.5));
#3976=CARTESIAN_POINT('',(-0.31,-0.9,2.5));
#3977=CARTESIAN_POINT('Origin',(0.,-0.9,2.5));
#3978=CARTESIAN_POINT('',(-0.31,-0.5,2.5));
#3979=CARTESIAN_POINT('',(-0.31,-1.,2.5));
#3980=CARTESIAN_POINT('Origin',(0.,-0.5,2.5));
#3981=CARTESIAN_POINT('Origin',(0.,-1.,2.5));
#3982=CARTESIAN_POINT('',(-0.31,0.5,2.5));
#3983=CARTESIAN_POINT('Origin',(0.,0.5,2.5));
#3984=CARTESIAN_POINT('',(-0.31,0.9,2.5));
#3985=CARTESIAN_POINT('',(-0.31,-1.,2.5));
#3986=CARTESIAN_POINT('Origin',(0.,0.9,2.5));
#3987=CARTESIAN_POINT('Origin',(0.,0.5,1.9));
#3988=CARTESIAN_POINT('',(0.7,0.5,3.3));
#3989=CARTESIAN_POINT('',(0.7,0.5,0.5));
#3990=CARTESIAN_POINT('',(-0.7,0.5,3.3));
#3991=CARTESIAN_POINT('',(0.7,0.5,3.3));
#3992=CARTESIAN_POINT('',(-0.7,0.5,3.3));
#3993=CARTESIAN_POINT('Origin',(0.7,0.5,3.3));
#3994=CARTESIAN_POINT('',(0.7,0.9,3.3));
#3995=CARTESIAN_POINT('',(0.7,0.9,0.5));
#3996=CARTESIAN_POINT('',(0.7,0.5,3.3));
#3997=CARTESIAN_POINT('Origin',(-0.7,0.5,0.5));
#3998=CARTESIAN_POINT('',(-0.7,0.9,3.3));
#3999=CARTESIAN_POINT('',(-0.7,0.5,3.3));
#4000=CARTESIAN_POINT('',(-0.7,0.9,3.3));
#4001=CARTESIAN_POINT('Origin',(-0.7,0.5,3.3));
#4002=CARTESIAN_POINT('',(0.7,0.9,3.3));
#4003=CARTESIAN_POINT('Origin',(0.,0.9,1.9));
#4004=CARTESIAN_POINT('Origin',(0.,-0.9,1.9));
#4005=CARTESIAN_POINT('',(0.7,-0.9,3.3));
#4006=CARTESIAN_POINT('',(0.7,-0.9,0.5));
#4007=CARTESIAN_POINT('',(-0.7,-0.9,3.3));
#4008=CARTESIAN_POINT('',(0.7,-0.9,3.3));
#4009=CARTESIAN_POINT('',(-0.7,-0.9,3.3));
#4010=CARTESIAN_POINT('Origin',(0.7,-0.9,3.3));
#4011=CARTESIAN_POINT('',(0.7,-0.5,3.3));
#4012=CARTESIAN_POINT('',(0.7,-0.5,0.5));
#4013=CARTESIAN_POINT('',(0.7,-0.9,3.3));
#4014=CARTESIAN_POINT('Origin',(-0.7,-0.9,0.5));
#4015=CARTESIAN_POINT('',(-0.7,-0.5,3.3));
#4016=CARTESIAN_POINT('',(-0.7,-0.9,3.3));
#4017=CARTESIAN_POINT('',(-0.7,-0.5,3.3));
#4018=CARTESIAN_POINT('Origin',(-0.7,-0.9,3.3));
#4019=CARTESIAN_POINT('',(0.7,-0.5,3.3));
#4020=CARTESIAN_POINT('Origin',(0.,-0.5,1.9));
#4021=CARTESIAN_POINT('Origin',(11.,-1.25,0.));
#4022=CARTESIAN_POINT('',(11.,-1.25,0.));
#4023=CARTESIAN_POINT('',(11.,-1.25,0.));
#4024=CARTESIAN_POINT('',(11.,-1.25,0.));
#4025=CARTESIAN_POINT('Origin',(-2.,-1.25,0.));
#4026=CARTESIAN_POINT('',(-2.,-1.25,0.));
#4027=CARTESIAN_POINT('',(-2.,-1.25,0.));
#4028=CARTESIAN_POINT('',(-2.,-1.25,0.));
#4029=CARTESIAN_POINT('Origin',(-2.,1.25,0.));
#4030=CARTESIAN_POINT('',(-2.,1.25,0.));
#4031=CARTESIAN_POINT('Origin',(4.5,0.,0.));
#4756=UNCERTAINTY_MEASURE_WITH_UNIT(LENGTH_MEASURE(0.001),#4792,
'DISTANCE_ACCURACY_VALUE',
'Maximum model space distance between geometric entities at asserted c
onnectivities');
#4772=UNCERTAINTY_MEASURE_WITH_UNIT(LENGTH_MEASURE(0.001),#4792,
'DISTANCE_ACCURACY_VALUE',
'Maximum model space distance between geometric entities at asserted c
onnectivities');
#4775=(
GEOMETRIC_REPRESENTATION_CONTEXT(3)
GLOBAL_UNCERTAINTY_ASSIGNED_CONTEXT((#4756))
GLOBAL_UNIT_ASSIGNED_CONTEXT((#4792,#4794,#4795))
REPRESENTATION_CONTEXT('','3D')
);
#4791=(
GEOMETRIC_REPRESENTATION_CONTEXT(3)
GLOBAL_UNCERTAINTY_ASSIGNED_CONTEXT((#4772))
GLOBAL_UNIT_ASSIGNED_CONTEXT((#4792,#4794,#4795))
REPRESENTATION_CONTEXT('','3D')
);
#4792=(
LENGTH_UNIT()
NAMED_UNIT(*)
SI_UNIT(.CENTI.,.METRE.)
);
#4794=(
NAMED_UNIT(*)
PLANE_ANGLE_UNIT()
SI_UNIT($,.RADIAN.)
);
#4795=(
NAMED_UNIT(*)
SI_UNIT($,.STERADIAN.)
SOLID_ANGLE_UNIT()
);
#4798=SHAPE_DEFINITION_REPRESENTATION(#4816,#4862);
#4816=PRODUCT_DEFINITION_SHAPE('',$,#4881);
#4862=SHAPE_REPRESENTATION('',(#2789),#4775);
#4878=PRODUCT_DEFINITION_CONTEXT('part definition',#4934,'design');
#4881=PRODUCT_DEFINITION('Twenty-five millimetre clamp base',
'Twenty-five millimetre clamp base',#4899,#4878);
#4899=PRODUCT_DEFINITION_FORMATION('',$,#4938);
#4934=APPLICATION_CONTEXT(
'Core Data for Automotive Mechanical Design Process');
#4935=PRODUCT_CONTEXT('part definition',#4934,'mechanical');
#4938=PRODUCT('Twenty-five millimetre clamp base',
'Twenty-five millimetre clamp base','Twenty-five millimetre clamp base',
(#4935));
#4996=COLOUR_RGB('Dark Blue',0.08,0.2,0.34);
#4997=FILL_AREA_STYLE_COLOUR('',#4996);
#4998=FILL_AREA_STYLE('',(#4997));
#4999=SURFACE_STYLE_FILL_AREA(#4998);
#5000=SURFACE_SIDE_STYLE('',(#4999));
#5001=SURFACE_STYLE_USAGE(.BOTH.,#5000);
#5002=PRESENTATION_STYLE_ASSIGNMENT((#5001));
ENDSEC;
END-ISO-10303-21;
